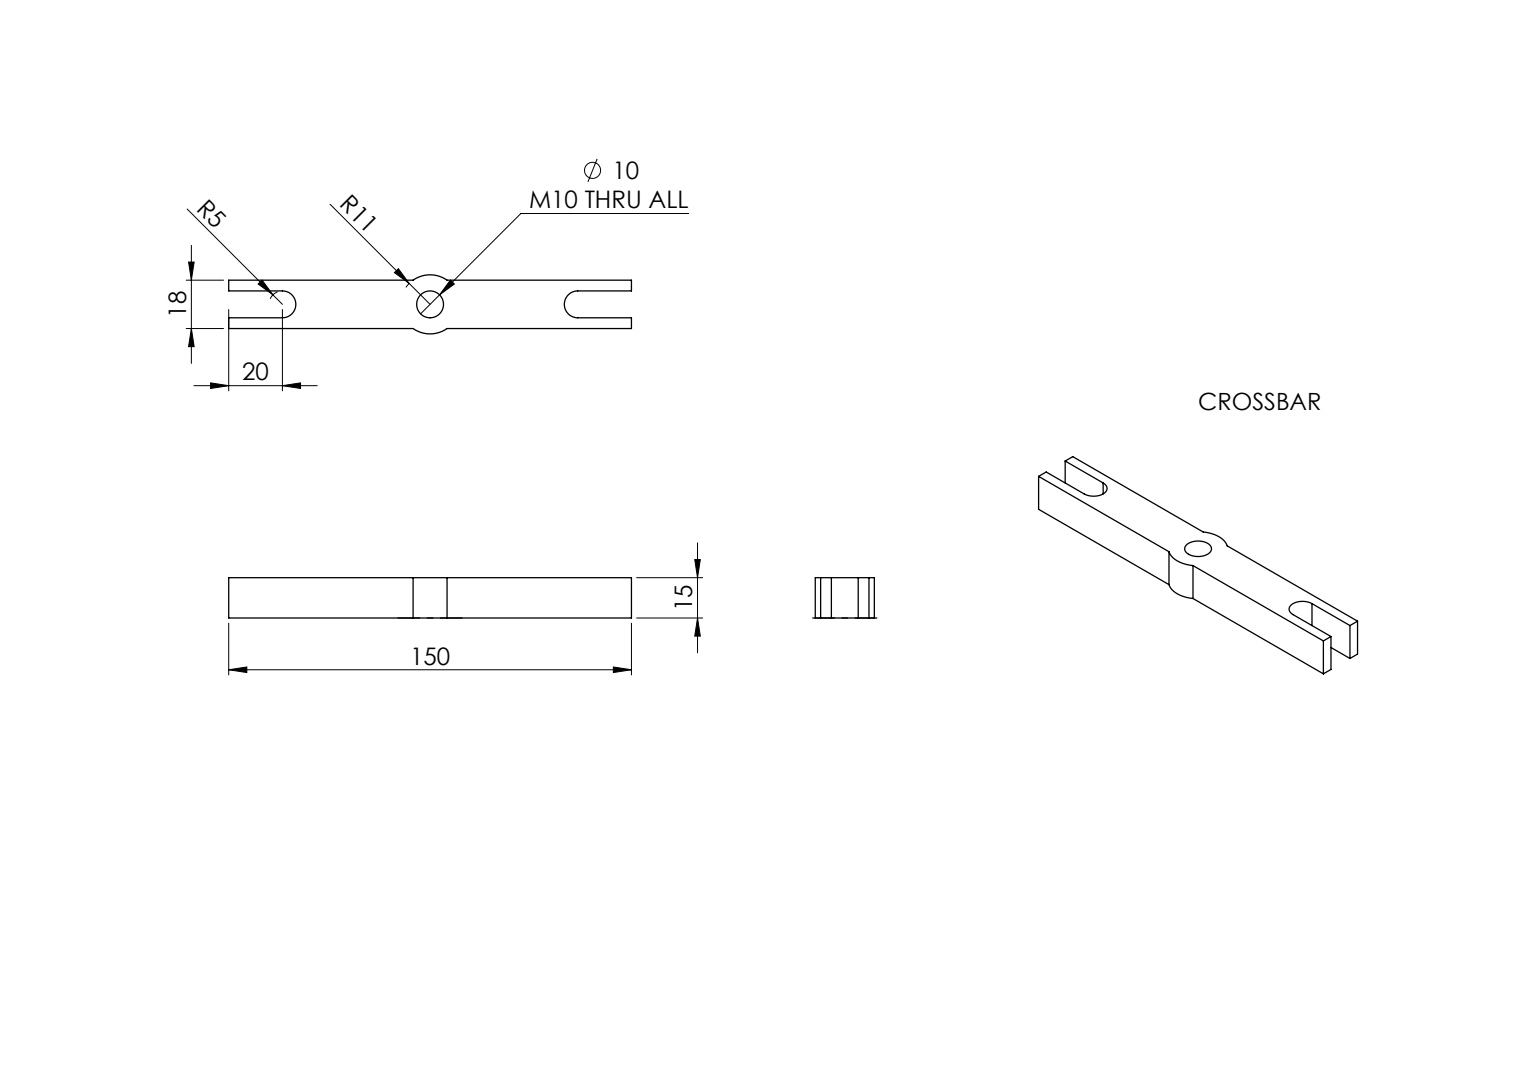
ISO-10303-21;
HEADER;
FILE_DESCRIPTION (('STEP AP214'),
    '1' );
FILE_NAME ('crossbar.step',
    '2026-10-25T05:52:03',
    ( '' ),
    ( '' ),
    'SwSTEP 2.0',
    'SolidWorks 2026',
    '' );
FILE_SCHEMA (( 'AUTOMOTIVE_DESIGN' ));
ENDSEC;

DATA;
#93=MECHANICAL_DESIGN_GEOMETRIC_PRESENTATION_REPRESENTATION('',(#59644),#40104);
#150=CARTESIAN_POINT ( 'NONE',  ( 0.000000000000000000, 15.00000000000000000, 0.000000000000000000 ) ) ;
#164=CARTESIAN_POINT ( 'NONE',  ( 75.00000000000002842, 15.00000000000000000, -5.000000000000000000 ) ) ;
#180=CARTESIAN_POINT ( 'NONE',  ( 75.00000000000000000, 15.00000000000000000, 8.999999999999998224 ) ) ;
#263=ORIENTED_EDGE ( 'NONE', *, *, #11129, .F. ) ;
#343=ORIENTED_EDGE ( 'NONE', *, *, #36170, .F. ) ;
#477=ORIENTED_EDGE ( 'NONE', *, *, #63171, .F. ) ;
#566=PRODUCT_CONTEXT ( 'NONE', #44181, 'mechanical' ) ;
#726=SURFACE_SIDE_STYLE ('',( #44126 ) ) ;
#1131=EDGE_CURVE ( 'NONE', #61397, #19898, #8913, .T. ) ;
#1258=VERTEX_POINT ( 'NONE', #48750 ) ;
#1307=DIRECTION ( 'NONE',  ( 0.000000000000000000, 0.000000000000000000, 1.000000000000000000 ) ) ;
#1344=DIRECTION ( 'NONE',  ( -1.000000000000000000, -0.000000000000000000, -0.000000000000000000 ) ) ;
#1422=LINE ( 'NONE', #21021, #18188 ) ;
#1774=VECTOR ( 'NONE', #54158, 1000.000000000000000 ) ;
#1820=AXIS2_PLACEMENT_3D ( 'NONE', #30255, #49878, #35415 ) ;
#1821=AXIS2_PLACEMENT_3D ( 'NONE', #44111, #19357, #38655 ) ;
#1868=CARTESIAN_POINT ( 'NONE',  ( 75.00000000000002842, 15.00000000000000000, -5.000000000000000000 ) ) ;
#1891=DIRECTION ( 'NONE',  ( -0.000000000000000000, -1.000000000000000000, -0.000000000000000000 ) ) ;
#1911=EDGE_CURVE ( 'NONE', #45549, #35107, #10129, .T. ) ;
#2018=DIRECTION ( 'NONE',  ( 0.000000000000000000, 0.000000000000000000, -1.000000000000000000 ) ) ;
#2144=CARTESIAN_POINT ( 'NONE',  ( 6.324555320336760822, 15.00000000000000000, 8.999999999999998224 ) ) ;
#2154=AXIS2_PLACEMENT_3D ( 'NONE', #31969, #51605, #37127 ) ;
#2168=ORIENTED_EDGE ( 'NONE', *, *, #7515, .F. ) ;
#2189=CARTESIAN_POINT ( 'NONE',  ( -75.00000000000001421, 15.00000000000000000, -9.000000000000001776 ) ) ;
#2419=DIRECTION ( 'NONE',  ( -1.000000000000000000, -0.000000000000000000, -0.000000000000000000 ) ) ;
#2521=EDGE_CURVE ( 'NONE', #37292, #8165, #8808, .T. ) ;
#2523=CARTESIAN_POINT ( 'NONE',  ( 0.000000000000000000, 0.000000000000000000, 0.000000000000000000 ) ) ;
#2751=FACE_OUTER_BOUND ( 'NONE', #28852, .T. ) ;
#3052=DIRECTION ( 'NONE',  ( 1.000000000000000000, -0.000000000000000000, -0.000000000000000000 ) ) ;
#3073=LINE ( 'NONE', #22370, #17419 ) ;
#3217=CARTESIAN_POINT ( 'NONE',  ( -75.00000000000002842, 15.00000000000000000, 5.000000000000000000 ) ) ;
#3275=VECTOR ( 'NONE', #5087, 1000.000000000000000 ) ;
#3526=DIRECTION ( 'NONE',  ( 1.000000000000000000, 0.000000000000000000, 0.000000000000000000 ) ) ;
#3683=LINE ( 'NONE', #52876, #59319 ) ;
#3701=DIRECTION ( 'NONE',  ( 0.000000000000000000, 0.000000000000000000, -1.000000000000000000 ) ) ;
#3724=CARTESIAN_POINT ( 'NONE',  ( 0.000000000000000000, 15.00000000000000000, 0.000000000000000000 ) ) ;
#3861=AXIS2_PLACEMENT_3D ( 'NONE', #23044, #42647, #37831 ) ;
#4005=EDGE_CURVE ( 'NONE', #32177, #5681, #30432, .T. ) ;
#4017=EDGE_CURVE ( 'NONE', #61397, #8313, #22859, .T. ) ;
#4135=VECTOR ( 'NONE', #36854, 1000.000000000000000 ) ;
#4205=ORIENTED_EDGE ( 'NONE', *, *, #4017, .F. ) ;
#4234=PLANE ( 'NONE',  #54494 ) ;
#4424=ORIENTED_EDGE ( 'NONE', *, *, #9501, .T. ) ;
#4477=ORIENTED_EDGE ( 'NONE', *, *, #9853, .F. ) ;
#4648=FACE_OUTER_BOUND ( 'NONE', #37201, .T. ) ;
#4801=ORIENTED_EDGE ( 'NONE', *, *, #10679, .F. ) ;
#5087=DIRECTION ( 'NONE',  ( -1.000000000000000000, -0.000000000000000000, -0.000000000000000000 ) ) ;
#5149=EDGE_CURVE ( 'NONE', #28986, #55261, #41034, .T. ) ;
#5151=CARTESIAN_POINT ( 'NONE',  ( 0.000000000000000000, 15.00000000000000000, 0.000000000000000000 ) ) ;
#5225=AXIS2_PLACEMENT_3D ( 'NONE', #12714, #42297, #61937 ) ;
#5300=CARTESIAN_POINT ( 'NONE',  ( -75.00000000000002842, 15.00000000000000000, -5.000000000000000000 ) ) ;
#5308=VERTEX_POINT ( 'NONE', #62260 ) ;
#5364=EDGE_CURVE ( 'NONE', #32593, #49211, #46190, .T. ) ;
#5608=VECTOR ( 'NONE', #49659, 1000.000000000000000 ) ;
#5626=EDGE_CURVE ( 'NONE', #47522, #36723, #20723, .T. ) ;
#5681=VERTEX_POINT ( 'NONE', #11056 ) ;
#5688=ORIENTED_EDGE ( 'NONE', *, *, #24345, .F. ) ;
#5744=AXIS2_PLACEMENT_3D ( 'NONE', #48462, #49087, #39429 ) ;
#5784=EDGE_LOOP ( 'NONE', ( #54539, #7926, #8477, #60385 ) ) ;
#5805=CARTESIAN_POINT ( 'NONE',  ( -75.00000000000000000, 15.00000000000000000, 8.999999999999998224 ) ) ;
#5822=DIRECTION ( 'NONE',  ( 0.000000000000000000, 0.000000000000000000, 1.000000000000000000 ) ) ;
#5858=EDGE_LOOP ( 'NONE', ( #24339, #2168, #263, #56580 ) ) ;
#5978=VECTOR ( 'NONE', #17876, 1000.000000000000000 ) ;
#6116=AXIS2_PLACEMENT_3D ( 'NONE', #16506, #11988, #35494 ) ;
#6272=EDGE_CURVE ( 'NONE', #47088, #29634, #54076, .T. ) ;
#6365=LINE ( 'NONE', #60400, #57679 ) ;
#6390=LINE ( 'NONE', #55597, #29862 ) ;
#6391=EDGE_LOOP ( 'NONE', ( #33069, #16377, #9474, #4205 ) ) ;
#6429=DIRECTION ( 'NONE',  ( 0.000000000000000000, -1.000000000000000000, 0.000000000000000000 ) ) ;
#6510=DIRECTION ( 'NONE',  ( 0.000000000000000000, -1.000000000000000000, 0.000000000000000000 ) ) ;
#6581=CARTESIAN_POINT ( 'NONE',  ( 75.00000000000002842, 15.00000000000000000, 5.000000000000000000 ) ) ;
#6625=VECTOR ( 'NONE', #29553, 1000.000000000000000 ) ;
#6635=ORIENTED_EDGE ( 'NONE', *, *, #1911, .F. ) ;
#6907=DIRECTION ( 'NONE',  ( -1.000000000000000000, 0.000000000000000000, 0.000000000000000000 ) ) ;
#7158=VERTEX_POINT ( 'NONE', #47572 ) ;
#7165=DIRECTION ( 'NONE',  ( 0.000000000000000000, -1.000000000000000000, 0.000000000000000000 ) ) ;
#7515=EDGE_CURVE ( 'NONE', #8991, #14704, #1422, .T. ) ;
#7900=EDGE_CURVE ( 'NONE', #56115, #33543, #15104, .T. ) ;
#7926=ORIENTED_EDGE ( 'NONE', *, *, #13807, .F. ) ;
#7954=ORIENTED_EDGE ( 'NONE', *, *, #58672, .T. ) ;
#8165=VERTEX_POINT ( 'NONE', #32166 ) ;
#8171=PLANE ( 'NONE',  #2154 ) ;
#8226=DIRECTION ( 'NONE',  ( -1.000000000000000000, 0.000000000000000000, 0.000000000000000000 ) ) ;
#8313=VERTEX_POINT ( 'NONE', #9924 ) ;
#8330=ORIENTED_EDGE ( 'NONE', *, *, #25196, .T. ) ;
#8418=ORIENTED_EDGE ( 'NONE', *, *, #39340, .F. ) ;
#8477=ORIENTED_EDGE ( 'NONE', *, *, #59318, .F. ) ;
#8690=ORIENTED_EDGE ( 'NONE', *, *, #4017, .T. ) ;
#8755=EDGE_LOOP ( 'NONE', ( #42090, #4424, #49121, #32813 ) ) ;
#8808=LINE ( 'NONE', #37769, #20258 ) ;
#8853=FACE_OUTER_BOUND ( 'NONE', #34956, .T. ) ;
#8913=CIRCLE ( 'NONE', #58273, 4.999999999999999112 ) ;
#8991=VERTEX_POINT ( 'NONE', #46151 ) ;
#9169=( GEOMETRIC_REPRESENTATION_CONTEXT ( 3 ) GLOBAL_UNCERTAINTY_ASSIGNED_CONTEXT ( ( #63524 ) ) GLOBAL_UNIT_ASSIGNED_CONTEXT ( ( #59255, #44448, #54100 ) ) REPRESENTATION_CONTEXT ( 'NONE', 'WORKASPACE' ) );
#9174=CIRCLE ( 'NONE', #6116, 5.000000000000000000 ) ;
#9243=LINE ( 'NONE', #18890, #15569 ) ;
#9272=ORIENTED_EDGE ( 'NONE', *, *, #62021, .F. ) ;
#9387=CARTESIAN_POINT ( 'NONE',  ( 6.324555320336760822, 15.00000000000000000, 8.999999999999998224 ) ) ;
#9474=ORIENTED_EDGE ( 'NONE', *, *, #17743, .T. ) ;
#9501=EDGE_CURVE ( 'NONE', #34999, #36723, #10721, .T. ) ;
#9795=CARTESIAN_POINT ( 'NONE',  ( 55.00000000000002132, 15.00000000000000000, 0.000000000000000000 ) ) ;
#9853=EDGE_CURVE ( 'NONE', #24525, #28986, #23225, .T. ) ;
#9872=ORIENTED_EDGE ( 'NONE', *, *, #25196, .F. ) ;
#9924=CARTESIAN_POINT ( 'NONE',  ( 0.000000000000000000, 15.00000000000000000, 5.000000000000000000 ) ) ;
#9961=CARTESIAN_POINT ( 'NONE',  ( 0.000000000000000000, 15.00000000000000000, 0.000000000000000000 ) ) ;
#10016=ADVANCED_FACE ( 'NONE', ( #19653 ), #55032, .F. ) ;
#10039=ORIENTED_EDGE ( 'NONE', *, *, #7515, .T. ) ;
#10087=ORIENTED_EDGE ( 'NONE', *, *, #24861, .T. ) ;
#10109=ORIENTED_EDGE ( 'NONE', *, *, #46867, .F. ) ;
#10129=LINE ( 'NONE', #180, #26454 ) ;
#10143=ORIENTED_EDGE ( 'NONE', *, *, #5626, .T. ) ;
#10259=ORIENTED_EDGE ( 'NONE', *, *, #26003, .T. ) ;
#10412=DIRECTION ( 'NONE',  ( -0.000000000000000000, -1.000000000000000000, -0.000000000000000000 ) ) ;
#10420=CARTESIAN_POINT ( 'NONE',  ( -75.00000000000001421, 15.00000000000000000, -9.000000000000001776 ) ) ;
#10679=EDGE_CURVE ( 'NONE', #57284, #54893, #23658, .T. ) ;
#10721=LINE ( 'NONE', #25513, #27505 ) ;
#10998=ORIENTED_EDGE ( 'NONE', *, *, #18539, .T. ) ;
#11056=CARTESIAN_POINT ( 'NONE',  ( -55.00000000000002132, 15.00000000000000000, -5.000000000000000000 ) ) ;
#11129=EDGE_CURVE ( 'NONE', #1258, #8991, #49113, .T. ) ;
#11150=CIRCLE ( 'NONE', #25528, 5.000000000000000000 ) ;
#11187=DIRECTION ( 'NONE',  ( 0.000000000000000000, -1.000000000000000000, 0.000000000000000000 ) ) ;
#11309=EDGE_LOOP ( 'NONE', ( #34515, #37261, #46350, #54536 ) ) ;
#11440=FACE_OUTER_BOUND ( 'NONE', #51205, .T. ) ;
#11539=DIRECTION ( 'NONE',  ( 0.000000000000000000, 0.000000000000000000, 1.000000000000000000 ) ) ;
#11675=LINE ( 'NONE', #39989, #46329 ) ;
#11732=EDGE_LOOP ( 'NONE', ( #24675, #13816, #20138, #18472 ) ) ;
#11762=ORIENTED_EDGE ( 'NONE', *, *, #2521, .F. ) ;
#11871=LINE ( 'NONE', #56596, #27063 ) ;
#11904=DIRECTION ( 'NONE',  ( -0.000000000000000000, -1.000000000000000000, -0.000000000000000000 ) ) ;
#11910=ADVANCED_FACE ( 'NONE', ( #42379 ), #17315, .T. ) ;
#11988=DIRECTION ( 'NONE',  ( -0.000000000000000000, 1.000000000000000000, -0.000000000000000000 ) ) ;
#12108=FACE_OUTER_BOUND ( 'NONE', #52618, .T. ) ;
#12280=ORIENTED_EDGE ( 'NONE', *, *, #54650, .F. ) ;
#12365=ORIENTED_EDGE ( 'NONE', *, *, #4005, .T. ) ;
#12559=EDGE_CURVE ( 'NONE', #54893, #57064, #27831, .T. ) ;
#12573=DIRECTION ( 'NONE',  ( 0.000000000000000000, 0.000000000000000000, -1.000000000000000000 ) ) ;
#12714=CARTESIAN_POINT ( 'NONE',  ( -55.00000000000002132, 0.000000000000000000, 0.000000000000000000 ) ) ;
#12872=CARTESIAN_POINT ( 'NONE',  ( -55.00000000000002132, 15.00000000000000000, 0.000000000000000000 ) ) ;
#12927=DIRECTION ( 'NONE',  ( 0.000000000000000000, 0.000000000000000000, 1.000000000000000000 ) ) ;
#12975=ORIENTED_EDGE ( 'NONE', *, *, #12559, .F. ) ;
#12976=DIRECTION ( 'NONE',  ( 1.000000000000000000, 0.000000000000000000, 0.000000000000000000 ) ) ;
#13083=ORIENTED_EDGE ( 'NONE', *, *, #55852, .F. ) ;
#13100=( LENGTH_UNIT ( ) NAMED_UNIT ( * ) SI_UNIT ( .MILLI., .METRE. ) );
#13235=CARTESIAN_POINT ( 'NONE',  ( -75.00000000000000000, 0.000000000000000000, 8.999999999999998224 ) ) ;
#13300=ORIENTED_EDGE ( 'NONE', *, *, #7900, .T. ) ;
#13340=PLANE ( 'NONE',  #59479 ) ;
#13356=CARTESIAN_POINT ( 'NONE',  ( -75.00000000000000000, 15.00000000000000000, 8.999999999999998224 ) ) ;
#13468=ADVANCED_FACE ( 'NONE', ( #37030 ), #22874, .T. ) ;
#13484=FACE_BOUND ( 'NONE', #40670, .T. ) ;
#13547=VERTEX_POINT ( 'NONE', #42467 ) ;
#13670=ORIENTED_EDGE ( 'NONE', *, *, #34124, .F. ) ;
#13807=EDGE_CURVE ( 'NONE', #1258, #57064, #57911, .T. ) ;
#13816=ORIENTED_EDGE ( 'NONE', *, *, #5149, .F. ) ;
#13817=DIRECTION ( 'NONE',  ( 0.000000000000000000, 0.000000000000000000, 1.000000000000000000 ) ) ;
#13856=ORIENTED_EDGE ( 'NONE', *, *, #42939, .F. ) ;
#13882=CARTESIAN_POINT ( 'NONE',  ( -75.00000000000000000, 15.00000000000000000, 8.999999999999998224 ) ) ;
#13919=DIRECTION ( 'NONE',  ( 1.000000000000000000, 0.000000000000000000, 0.000000000000000000 ) ) ;
#14074=ORIENTED_EDGE ( 'NONE', *, *, #18539, .F. ) ;
#14144=EDGE_CURVE ( 'NONE', #8313, #16398, #11150, .T. ) ;
#14157=ORIENTED_EDGE ( 'NONE', *, *, #37324, .F. ) ;
#14189=VECTOR ( 'NONE', #3052, 1000.000000000000000 ) ;
#14234=ADVANCED_FACE ( 'NONE', ( #8853 ), #28470, .F. ) ;
#14236=ORIENTED_EDGE ( 'NONE', *, *, #34954, .F. ) ;
#14305=STYLED_ITEM ( 'NONE', ( #19692 ), #24770 ) ;
#14412=DIRECTION ( 'NONE',  ( 0.000000000000000000, -1.000000000000000000, 0.000000000000000000 ) ) ;
#14445=ADVANCED_FACE ( 'NONE', ( #4648 ), #63520, .T. ) ;
#14618=UNCERTAINTY_MEASURE_WITH_UNIT (LENGTH_MEASURE( 1.000000000000000082E-05 ), #20010, 'distance_accuracy_value', 'NONE');
#14661=ORIENTED_EDGE ( 'NONE', *, *, #1911, .T. ) ;
#14704=VERTEX_POINT ( 'NONE', #27767 ) ;
#14783=PRODUCT_DEFINITION_SHAPE ( 'NONE', 'NONE',  #53574 ) ;
#14797=ORIENTED_EDGE ( 'NONE', *, *, #24861, .F. ) ;
#14808=ORIENTED_EDGE ( 'NONE', *, *, #43189, .T. ) ;
#14951=CARTESIAN_POINT ( 'NONE',  ( -55.00000000000002132, 15.00000000000000000, -5.000000000000000000 ) ) ;
#15006=VECTOR ( 'NONE', #3526, 1000.000000000000000 ) ;
#15104=CIRCLE ( 'NONE', #1820, 11.00000000000000000 ) ;
#15481=CARTESIAN_POINT ( 'NONE',  ( 0.000000000000000000, 15.00000000000000000, 0.000000000000000000 ) ) ;
#15569=VECTOR ( 'NONE', #33688, 1000.000000000000000 ) ;
#15748=CARTESIAN_POINT ( 'NONE',  ( -75.00000000000000000, 0.000000000000000000, 8.999999999999998224 ) ) ;
#15753=DIRECTION ( 'NONE',  ( 0.000000000000000000, 1.000000000000000000, 0.000000000000000000 ) ) ;
#15757=ORIENTED_EDGE ( 'NONE', *, *, #54792, .T. ) ;
#15761=EDGE_CURVE ( 'NONE', #55261, #54893, #45335, .T. ) ;
#15836=ORIENTED_EDGE ( 'NONE', *, *, #56237, .F. ) ;
#15970=ORIENTED_EDGE ( 'NONE', *, *, #1131, .T. ) ;
#15986=DIRECTION ( 'NONE',  ( -0.000000000000000000, 1.000000000000000000, -0.000000000000000000 ) ) ;
#16016=CARTESIAN_POINT ( 'NONE',  ( -75.00000000000002842, 15.00000000000000000, -5.000000000000000000 ) ) ;
#16270=PLANE ( 'NONE',  #62054 ) ;
#16377=ORIENTED_EDGE ( 'NONE', *, *, #62021, .T. ) ;
#16398=VERTEX_POINT ( 'NONE', #41056 ) ;
#16506=CARTESIAN_POINT ( 'NONE',  ( 0.000000000000000000, 15.00000000000000000, 0.000000000000000000 ) ) ;
#16597=LINE ( 'NONE', #2144, #4135 ) ;
#16603=DIRECTION ( 'NONE',  ( 7.709882115452476194E-16, 0.000000000000000000, -1.000000000000000000 ) ) ;
#16845=ADVANCED_FACE ( 'NONE', ( #59014 ), #21621, .F. ) ;
#16858=CARTESIAN_POINT ( 'NONE',  ( -6.324555320336756381, 0.000000000000000000, -9.000000000000001776 ) ) ;
#16869=DIRECTION ( 'NONE',  ( 0.000000000000000000, 0.000000000000000000, 1.000000000000000000 ) ) ;
#16955=AXIS2_PLACEMENT_3D ( 'NONE', #37433, #62204, #57065 ) ;
#16959=DIRECTION ( 'NONE',  ( 1.000000000000000000, 0.000000000000000000, -0.000000000000000000 ) ) ;
#17205=EDGE_CURVE ( 'NONE', #57064, #14704, #51349, .T. ) ;
#17257=VERTEX_POINT ( 'NONE', #59804 ) ;
#17315=PLANE ( 'NONE',  #34702 ) ;
#17325=ORIENTED_EDGE ( 'NONE', *, *, #11129, .T. ) ;
#17381=ADVANCED_FACE ( 'NONE', ( #2751 ), #47436, .T. ) ;
#17387=EDGE_CURVE ( 'NONE', #28986, #57284, #3073, .T. ) ;
#17419=VECTOR ( 'NONE', #22690, 1000.000000000000000 ) ;
#17440=ORIENTED_EDGE ( 'NONE', *, *, #59318, .T. ) ;
#17459=VECTOR ( 'NONE', #41732, 1000.000000000000000 ) ;
#17506=CARTESIAN_POINT ( 'NONE',  ( -75.00000000000000000, 0.000000000000000000, 8.999999999999998224 ) ) ;
#17594=VECTOR ( 'NONE', #47304, 1000.000000000000000 ) ;
#17743=EDGE_CURVE ( 'NONE', #16398, #8313, #9174, .T. ) ;
#17751=DIRECTION ( 'NONE',  ( 1.000000000000000000, 0.000000000000000000, 0.000000000000000000 ) ) ;
#17808=CARTESIAN_POINT ( 'NONE',  ( -75.00000000000002842, 15.00000000000000000, 5.000000000000000000 ) ) ;
#17876=DIRECTION ( 'NONE',  ( 7.709882115452476194E-16, 0.000000000000000000, -1.000000000000000000 ) ) ;
#17936=DIRECTION ( 'NONE',  ( 1.000000000000000000, 0.000000000000000000, 0.000000000000000000 ) ) ;
#18188=VECTOR ( 'NONE', #31287, 1000.000000000000000 ) ;
#18368=FACE_OUTER_BOUND ( 'NONE', #11309, .T. ) ;
#18410=VECTOR ( 'NONE', #1344, 1000.000000000000000 ) ;
#18456=AXIS2_PLACEMENT_3D ( 'NONE', #52894, #28127, #3701 ) ;
#18472=ORIENTED_EDGE ( 'NONE', *, *, #10679, .T. ) ;
#18539=EDGE_CURVE ( 'NONE', #17257, #47088, #56236, .T. ) ;
#18621=CARTESIAN_POINT ( 'NONE',  ( -75.00000000000002842, 15.00000000000000000, -5.000000000000000000 ) ) ;
#18677=DIRECTION ( 'NONE',  ( 0.000000000000000000, 0.000000000000000000, -1.000000000000000000 ) ) ;
#18779=DIRECTION ( 'NONE',  ( -1.000000000000000000, 0.000000000000000000, -0.000000000000000000 ) ) ;
#18875=PRODUCT ( 'crossbar', 'crossbar', '', ( #566 ) ) ;
#18890=CARTESIAN_POINT ( 'NONE',  ( -75.00000000000000000, 0.000000000000000000, 8.999999999999998224 ) ) ;
#18963=EDGE_CURVE ( 'NONE', #7158, #24525, #16597, .T. ) ;
#19009=DIRECTION ( 'NONE',  ( 1.000000000000000000, 0.000000000000000000, -0.000000000000000000 ) ) ;
#19045=VECTOR ( 'NONE', #12976, 1000.000000000000000 ) ;
#19129=AXIS2_PLACEMENT_3D ( 'NONE', #2189, #41701, #16959 ) ;
#19188=ORIENTED_EDGE ( 'NONE', *, *, #39340, .T. ) ;
#19357=DIRECTION ( 'NONE',  ( 0.000000000000000000, 0.000000000000000000, -1.000000000000000000 ) ) ;
#19373=( NAMED_UNIT ( * ) PLANE_ANGLE_UNIT ( ) SI_UNIT ( $, .RADIAN. ) );
#19397=ADVANCED_FACE ( 'NONE', ( #29068 ), #59308, .T. ) ;
#19653=FACE_OUTER_BOUND ( 'NONE', #6391, .T. ) ;
#19692=PRESENTATION_STYLE_ASSIGNMENT (( #29653 ) ) ;
#19745=DIRECTION ( 'NONE',  ( -0.000000000000000000, -1.000000000000000000, -0.000000000000000000 ) ) ;
#19765=ORIENTED_EDGE ( 'NONE', *, *, #59330, .T. ) ;
#19793=VERTEX_POINT ( 'NONE', #53451 ) ;
#19898=VERTEX_POINT ( 'NONE', #54409 ) ;
#20010=( LENGTH_UNIT ( ) NAMED_UNIT ( * ) SI_UNIT ( .MILLI., .METRE. ) );
#20138=ORIENTED_EDGE ( 'NONE', *, *, #17387, .T. ) ;
#20258=VECTOR ( 'NONE', #42585, 1000.000000000000000 ) ;
#20336=SHAPE_REPRESENTATION_RELATIONSHIP ( 'NONE' , 'NONE' ,  #21293, #24770 ) ;
#20432=VECTOR ( 'NONE', #6429, 1000.000000000000000 ) ;
#20535=AXIS2_PLACEMENT_3D ( 'NONE', #150, #19745, #58988 ) ;
#20723=LINE ( 'NONE', #10420, #1774 ) ;
#21021=CARTESIAN_POINT ( 'NONE',  ( 55.00000000000002132, 15.00000000000000000, -5.000000000000000000 ) ) ;
#21184=ORIENTED_EDGE ( 'NONE', *, *, #34954, .T. ) ;
#21202=CARTESIAN_POINT ( 'NONE',  ( -75.00000000000000000, 15.00000000000000000, 8.999999999999998224 ) ) ;
#21219=DIRECTION ( 'NONE',  ( 7.709882115452476194E-16, -0.000000000000000000, 1.000000000000000000 ) ) ;
#21287=ORIENTED_EDGE ( 'NONE', *, *, #9501, .F. ) ;
#21293=SHAPE_REPRESENTATION ( 'crossbar', ( #43054 ), #21498 ) ;
#21357=VECTOR ( 'NONE', #6907, 1000.000000000000000 ) ;
#21440=ORIENTED_EDGE ( 'NONE', *, *, #22095, .T. ) ;
#21498=( GEOMETRIC_REPRESENTATION_CONTEXT ( 3 ) GLOBAL_UNCERTAINTY_ASSIGNED_CONTEXT ( ( #14618 ) ) GLOBAL_UNIT_ASSIGNED_CONTEXT ( ( #20010, #19373, #58929 ) ) REPRESENTATION_CONTEXT ( 'NONE', 'WORKASPACE' ) );
#21621=CYLINDRICAL_SURFACE ( 'NONE', #27642, 5.000000000000000000 ) ;
#21637=CARTESIAN_POINT ( 'NONE',  ( -55.00000000000002132, 15.00000000000000000, 5.000000000000000000 ) ) ;
#21838=DIRECTION ( 'NONE',  ( 0.000000000000000000, 1.000000000000000000, 0.000000000000000000 ) ) ;
#21947=ADVANCED_FACE ( 'NONE', ( #11440 ), #55200, .F. ) ;
#21950=FACE_OUTER_BOUND ( 'NONE', #60332, .T. ) ;
#22095=EDGE_CURVE ( 'NONE', #8165, #34549, #56581, .T. ) ;
#22107=PLANE ( 'NONE',  #19129 ) ;
#22137=CARTESIAN_POINT ( 'NONE',  ( -75.00000000000001421, 0.000000000000000000, -9.000000000000001776 ) ) ;
#22211=DIRECTION ( 'NONE',  ( 1.000000000000000000, -0.000000000000000000, -0.000000000000000000 ) ) ;
#22271=DIRECTION ( 'NONE',  ( 0.000000000000000000, -0.000000000000000000, -1.000000000000000000 ) ) ;
#22370=CARTESIAN_POINT ( 'NONE',  ( 75.00000000000000000, 15.00000000000000000, 8.999999999999998224 ) ) ;
#22384=LINE ( 'NONE', #51655, #47156 ) ;
#22390=ORIENTED_EDGE ( 'NONE', *, *, #22398, .T. ) ;
#22398=EDGE_CURVE ( 'NONE', #58460, #19793, #11675, .T. ) ;
#22429=FACE_OUTER_BOUND ( 'NONE', #8755, .T. ) ;
#22558=MECHANICAL_DESIGN_GEOMETRIC_PRESENTATION_REPRESENTATION('',(#14305),#9169);
#22650=LINE ( 'NONE', #17506, #19045 ) ;
#22690=DIRECTION ( 'NONE',  ( -0.000000000000000000, -1.000000000000000000, -0.000000000000000000 ) ) ;
#22831=LINE ( 'NONE', #18621, #3275 ) ;
#22859=LINE ( 'NONE', #27978, #26312 ) ;
#22874=PLANE ( 'NONE',  #53254 ) ;
#22920=FACE_OUTER_BOUND ( 'NONE', #43636, .T. ) ;
#23028=DIRECTION ( 'NONE',  ( -1.000000000000000000, 0.000000000000000000, -0.000000000000000000 ) ) ;
#23044=CARTESIAN_POINT ( 'NONE',  ( 0.000000000000000000, 15.00000000000000000, 0.000000000000000000 ) ) ;
#23071=( NAMED_UNIT ( * ) PLANE_ANGLE_UNIT ( ) SI_UNIT ( $, .RADIAN. ) );
#23225=LINE ( 'NONE', #13882, #34654 ) ;
#23288=VECTOR ( 'NONE', #16603, 1000.000000000000000 ) ;
#23412=CARTESIAN_POINT ( 'NONE',  ( -75.00000000000002842, 15.00000000000000000, -5.000000000000000000 ) ) ;
#23425=VECTOR ( 'NONE', #30375, 1000.000000000000000 ) ;
#23604=AXIS2_PLACEMENT_3D ( 'NONE', #36302, #31786, #45632 ) ;
#23658=LINE ( 'NONE', #62893, #5978 ) ;
#23669=ORIENTED_EDGE ( 'NONE', *, *, #59330, .F. ) ;
#23825=CYLINDRICAL_SURFACE ( 'NONE', #37129, 11.00000000000000000 ) ;
#24247=ORIENTED_EDGE ( 'NONE', *, *, #4005, .F. ) ;
#24339=ORIENTED_EDGE ( 'NONE', *, *, #17205, .T. ) ;
#24345=EDGE_CURVE ( 'NONE', #29634, #34999, #30937, .T. ) ;
#24471=ORIENTED_EDGE ( 'NONE', *, *, #37324, .T. ) ;
#24524=FILL_AREA_STYLE ('',( #58306 ) ) ;
#24525=VERTEX_POINT ( 'NONE', #9387 ) ;
#24675=ORIENTED_EDGE ( 'NONE', *, *, #15761, .F. ) ;
#24770=ADVANCED_BREP_SHAPE_REPRESENTATION ( '', ( #29015, #43054 ), #21498 ) ;
#24861=EDGE_CURVE ( 'NONE', #32177, #8165, #42463, .T. ) ;
#25136=ORIENTED_EDGE ( 'NONE', *, *, #54792, .F. ) ;
#25196=EDGE_CURVE ( 'NONE', #36723, #26676, #9243, .T. ) ;
#25352=CLOSED_SHELL ( 'NONE', ( #10016, #19397, #29448, #21947, #26816, #32085, #40968, #34918, #45695, #28741, #14234, #51439, #17381, #30357, #29838, #44373, #11910, #13468, #16845, #14445, #55014 ) ) ;
#25382=ORIENTED_EDGE ( 'NONE', *, *, #24345, .T. ) ;
#25395=DIRECTION ( 'NONE',  ( 7.709882115452476194E-16, -0.000000000000000000, 1.000000000000000000 ) ) ;
#25404=EDGE_CURVE ( 'NONE', #34999, #13547, #6365, .T. ) ;
#25513=CARTESIAN_POINT ( 'NONE',  ( -75.00000000000001421, 0.000000000000000000, -9.000000000000001776 ) ) ;
#25528=AXIS2_PLACEMENT_3D ( 'NONE', #3724, #31473, #51114 ) ;
#25545=EDGE_LOOP ( 'NONE', ( #15970, #60870 ) ) ;
#25767=CARTESIAN_POINT ( 'NONE',  ( -75.00000000000001421, 15.00000000000000000, -9.000000000000001776 ) ) ;
#26003=EDGE_CURVE ( 'NONE', #35107, #17257, #54196, .T. ) ;
#26125=CARTESIAN_POINT ( 'NONE',  ( 75.00000000000002842, 15.00000000000000000, 5.000000000000000000 ) ) ;
#26184=ORIENTED_EDGE ( 'NONE', *, *, #49243, .T. ) ;
#26236=DIRECTION ( 'NONE',  ( -7.709882115452477180E-16, 0.000000000000000000, 1.000000000000000000 ) ) ;
#26312=VECTOR ( 'NONE', #42768, 1000.000000000000000 ) ;
#26403=VECTOR ( 'NONE', #11904, 1000.000000000000000 ) ;
#26454=VECTOR ( 'NONE', #43579, 1000.000000000000000 ) ;
#26676=VERTEX_POINT ( 'NONE', #27009 ) ;
#26680=PRODUCT_DEFINITION_FORMATION_WITH_SPECIFIED_SOURCE ( 'ANY', '', #18875, .NOT_KNOWN. ) ;
#26771=AXIS2_PLACEMENT_3D ( 'NONE', #30746, #50681, #26236 ) ;
#26806=EDGE_CURVE ( 'NONE', #5681, #42641, #22831, .T. ) ;
#26816=ADVANCED_FACE ( 'NONE', ( #13484, #57865 ), #29511, .F. ) ;
#26860=CARTESIAN_POINT ( 'NONE',  ( -75.00000000000001421, 15.00000000000000000, -9.000000000000001776 ) ) ;
#26967=ORIENTED_EDGE ( 'NONE', *, *, #22095, .F. ) ;
#27004=CARTESIAN_POINT ( 'NONE',  ( 75.00000000000000000, 0.000000000000000000, 8.999999999999998224 ) ) ;
#27009=CARTESIAN_POINT ( 'NONE',  ( -75.00000000000002842, 0.000000000000000000, -5.000000000000000000 ) ) ;
#27063=VECTOR ( 'NONE', #21219, 1000.000000000000000 ) ;
#27084=LINE ( 'NONE', #47953, #42835 ) ;
#27505=VECTOR ( 'NONE', #62939, 1000.000000000000000 ) ;
#27541=VECTOR ( 'NONE', #2419, 1000.000000000000000 ) ;
#27642=AXIS2_PLACEMENT_3D ( 'NONE', #9795, #6510, #2018 ) ;
#27665=DIRECTION ( 'NONE',  ( 0.000000000000000000, 1.000000000000000000, 0.000000000000000000 ) ) ;
#27767=CARTESIAN_POINT ( 'NONE',  ( 55.00000000000002132, -0.000000000000000000, -5.000000000000000000 ) ) ;
#27789=CARTESIAN_POINT ( 'NONE',  ( 75.00000000000002842, 15.00000000000000000, -5.000000000000000000 ) ) ;
#27831=LINE ( 'NONE', #61948, #31682 ) ;
#27978=CARTESIAN_POINT ( 'NONE',  ( 0.000000000000000000, 15.00000000000000000, 4.999999999999999112 ) ) ;
#28127=DIRECTION ( 'NONE',  ( -0.000000000000000000, -1.000000000000000000, -0.000000000000000000 ) ) ;
#28148=VECTOR ( 'NONE', #29409, 1000.000000000000000 ) ;
#28195=CARTESIAN_POINT ( 'NONE',  ( 0.000000000000000000, 0.000000000000000000, 0.000000000000000000 ) ) ;
#28470=PLANE ( 'NONE',  #61499 ) ;
#28704=ORIENTED_EDGE ( 'NONE', *, *, #25404, .T. ) ;
#28741=ADVANCED_FACE ( 'NONE', ( #22920 ), #4234, .F. ) ;
#28773=EDGE_CURVE ( 'NONE', #33543, #29634, #6390, .T. ) ;
#28779=EDGE_LOOP ( 'NONE', ( #11762, #14236, #62039, #10087 ) ) ;
#28838=CYLINDRICAL_SURFACE ( 'NONE', #5744, 5.000000000000000000 ) ;
#28852=EDGE_LOOP ( 'NONE', ( #30021, #31055, #30696, #22390 ) ) ;
#28986=VERTEX_POINT ( 'NONE', #37235 ) ;
#29015=MANIFOLD_SOLID_BREP ( 'AdvancedHole2', #25352 ) ;
#29068=FACE_OUTER_BOUND ( 'NONE', #37644, .T. ) ;
#29262=CARTESIAN_POINT ( 'NONE',  ( 55.00000000000002132, 0.000000000000000000, 5.000000000000000000 ) ) ;
#29409=DIRECTION ( 'NONE',  ( 0.000000000000000000, -1.000000000000000000, 0.000000000000000000 ) ) ;
#29448=ADVANCED_FACE ( 'NONE', ( #40697 ), #16270, .F. ) ;
#29491=CIRCLE ( 'NONE', #3861, 11.00000000000000000 ) ;
#29511=PLANE ( 'NONE',  #55525 ) ;
#29553=DIRECTION ( 'NONE',  ( 1.000000000000000000, 0.000000000000000000, 0.000000000000000000 ) ) ;
#29634=VERTEX_POINT ( 'NONE', #36841 ) ;
#29653=SURFACE_STYLE_USAGE ( .BOTH. , #726 ) ;
#29765=CARTESIAN_POINT ( 'NONE',  ( 75.00000000000000000, 15.00000000000000000, 8.999999999999998224 ) ) ;
#29838=ADVANCED_FACE ( 'NONE', ( #33585 ), #13340, .T. ) ;
#29862=VECTOR ( 'NONE', #1891, 1000.000000000000000 ) ;
#30021=ORIENTED_EDGE ( 'NONE', *, *, #56237, .T. ) ;
#30030=CARTESIAN_POINT ( 'NONE',  ( -75.00000000000000000, 15.00000000000000000, 8.999999999999998224 ) ) ;
#30057=CARTESIAN_POINT ( 'NONE',  ( 75.00000000000002842, 0.000000000000000000, -5.000000000000000000 ) ) ;
#30086=DIRECTION ( 'NONE',  ( -7.709882115452477180E-16, 0.000000000000000000, 1.000000000000000000 ) ) ;
#30255=CARTESIAN_POINT ( 'NONE',  ( 0.000000000000000000, 15.00000000000000000, 0.000000000000000000 ) ) ;
#30291=EDGE_LOOP ( 'NONE', ( #26967, #14797, #12365, #24471 ) ) ;
#30357=ADVANCED_FACE ( 'NONE', ( #18368 ), #23825, .T. ) ;
#30375=DIRECTION ( 'NONE',  ( -1.000000000000000000, -0.000000000000000000, -0.000000000000000000 ) ) ;
#30432=CIRCLE ( 'NONE', #58170, 5.000000000000000000 ) ;
#30576=DIRECTION ( 'NONE',  ( 0.000000000000000000, 0.000000000000000000, 1.000000000000000000 ) ) ;
#30594=ORIENTED_EDGE ( 'NONE', *, *, #55852, .T. ) ;
#30696=ORIENTED_EDGE ( 'NONE', *, *, #43189, .F. ) ;
#30711=DIRECTION ( 'NONE',  ( -0.000000000000000000, -1.000000000000000000, -0.000000000000000000 ) ) ;
#30746=CARTESIAN_POINT ( 'NONE',  ( 75.00000000000000000, 15.00000000000000000, 8.999999999999998224 ) ) ;
#30895=LINE ( 'NONE', #59864, #26403 ) ;
#30937=CIRCLE ( 'NONE', #40212, 11.00000000000000000 ) ;
#31055=ORIENTED_EDGE ( 'NONE', *, *, #18963, .T. ) ;
#31096=DIRECTION ( 'NONE',  ( 0.000000000000000000, 0.000000000000000000, 1.000000000000000000 ) ) ;
#31287=DIRECTION ( 'NONE',  ( 0.000000000000000000, -1.000000000000000000, 0.000000000000000000 ) ) ;
#31466=CARTESIAN_POINT ( 'NONE',  ( 0.000000000000000000, 0.000000000000000000, 0.000000000000000000 ) ) ;
#31473=DIRECTION ( 'NONE',  ( -0.000000000000000000, 1.000000000000000000, -0.000000000000000000 ) ) ;
#31511=EDGE_CURVE ( 'NONE', #8991, #45549, #51929, .T. ) ;
#31636=VECTOR ( 'NONE', #59988, 1000.000000000000000 ) ;
#31642=AXIS2_PLACEMENT_3D ( 'NONE', #48917, #39900, #30576 ) ;
#31676=ORIENTED_EDGE ( 'NONE', *, *, #47226, .F. ) ;
#31682=VECTOR ( 'NONE', #8226, 1000.000000000000000 ) ;
#31786=DIRECTION ( 'NONE',  ( -0.000000000000000000, -1.000000000000000000, -0.000000000000000000 ) ) ;
#31965=ORIENTED_EDGE ( 'NONE', *, *, #42939, .T. ) ;
#31969=CARTESIAN_POINT ( 'NONE',  ( -75.00000000000000000, 15.00000000000000000, 8.999999999999998224 ) ) ;
#32022=ORIENTED_EDGE ( 'NONE', *, *, #31511, .T. ) ;
#32085=ADVANCED_FACE ( 'NONE', ( #61197, #21950 ), #46074, .T. ) ;
#32166=CARTESIAN_POINT ( 'NONE',  ( -55.00000000000002132, 0.000000000000000000, 5.000000000000000000 ) ) ;
#32177=VERTEX_POINT ( 'NONE', #21637 ) ;
#32593=VERTEX_POINT ( 'NONE', #5805 ) ;
#32599=AXIS2_PLACEMENT_3D ( 'NONE', #56755, #56441, #16869 ) ;
#32601=FACE_OUTER_BOUND ( 'NONE', #37600, .T. ) ;
#32813=ORIENTED_EDGE ( 'NONE', *, *, #58672, .F. ) ;
#32979=DIRECTION ( 'NONE',  ( -0.000000000000000000, -1.000000000000000000, -0.000000000000000000 ) ) ;
#33069=ORIENTED_EDGE ( 'NONE', *, *, #61030, .F. ) ;
#33143=ORIENTED_EDGE ( 'NONE', *, *, #36170, .T. ) ;
#33287=DIRECTION ( 'NONE',  ( -0.000000000000000000, 1.000000000000000000, -0.000000000000000000 ) ) ;
#33532=FACE_OUTER_BOUND ( 'NONE', #60854, .T. ) ;
#33543=VERTEX_POINT ( 'NONE', #39297 ) ;
#33585=FACE_OUTER_BOUND ( 'NONE', #28779, .T. ) ;
#33603=ORIENTED_EDGE ( 'NONE', *, *, #26806, .T. ) ;
#33670=FACE_OUTER_BOUND ( 'NONE', #30291, .T. ) ;
#33688=DIRECTION ( 'NONE',  ( 7.709882115452476194E-16, -0.000000000000000000, 1.000000000000000000 ) ) ;
#33911=VECTOR ( 'NONE', #30711, 1000.000000000000000 ) ;
#34078=DIRECTION ( 'NONE',  ( 0.000000000000000000, -1.000000000000000000, 0.000000000000000000 ) ) ;
#34124=EDGE_CURVE ( 'NONE', #37292, #49211, #34724, .T. ) ;
#34233=CARTESIAN_POINT ( 'NONE',  ( -55.00000000000002132, 0.000000000000000000, -5.000000000000000000 ) ) ;
#34345=CARTESIAN_POINT ( 'NONE',  ( 0.000000000000000000, 15.00000000000000000, 0.000000000000000000 ) ) ;
#34515=ORIENTED_EDGE ( 'NONE', *, *, #28773, .F. ) ;
#34549=VERTEX_POINT ( 'NONE', #34233 ) ;
#34650=CIRCLE ( 'NONE', #32599, 11.00000000000000000 ) ;
#34654=VECTOR ( 'NONE', #57340, 1000.000000000000000 ) ;
#34702=AXIS2_PLACEMENT_3D ( 'NONE', #23412, #62656, #17936 ) ;
#34724=LINE ( 'NONE', #15748, #45142 ) ;
#34884=DIRECTION ( 'NONE',  ( 0.000000000000000000, 0.000000000000000000, 1.000000000000000000 ) ) ;
#34900=CARTESIAN_POINT ( 'NONE',  ( -75.00000000000002842, 0.000000000000000000, 5.000000000000000000 ) ) ;
#34918=ADVANCED_FACE ( 'NONE', ( #32601 ), #8171, .F. ) ;
#34954=EDGE_CURVE ( 'NONE', #5308, #37292, #51291, .T. ) ;
#34956=EDGE_LOOP ( 'NONE', ( #45657, #31965, #55754, #4477 ) ) ;
#34999=VERTEX_POINT ( 'NONE', #16858 ) ;
#35107=VERTEX_POINT ( 'NONE', #57690 ) ;
#35367=CARTESIAN_POINT ( 'NONE',  ( 75.00000000000002842, 15.00000000000000000, 5.000000000000000000 ) ) ;
#35415=DIRECTION ( 'NONE',  ( 0.000000000000000000, 0.000000000000000000, 1.000000000000000000 ) ) ;
#35494=DIRECTION ( 'NONE',  ( 0.000000000000000000, 0.000000000000000000, 1.000000000000000000 ) ) ;
#35824=AXIS2_PLACEMENT_3D ( 'NONE', #164, #34884, #54506 ) ;
#35889=DIRECTION ( 'NONE',  ( -1.000000000000000000, 0.000000000000000000, -7.709882115452477180E-16 ) ) ;
#36159=ORIENTED_EDGE ( 'NONE', *, *, #59338, .F. ) ;
#36170=EDGE_CURVE ( 'NONE', #5308, #32593, #11871, .T. ) ;
#36302=CARTESIAN_POINT ( 'NONE',  ( 55.00000000000002132, 0.000000000000000000, 0.000000000000000000 ) ) ;
#36422=CARTESIAN_POINT ( 'NONE',  ( 0.000000000000000000, 0.000000000000000000, 0.000000000000000000 ) ) ;
#36508=CIRCLE ( 'NONE', #45742, 11.00000000000000000 ) ;
#36584=CARTESIAN_POINT ( 'NONE',  ( -75.00000000000001421, 15.00000000000000000, -9.000000000000001776 ) ) ;
#36723=VERTEX_POINT ( 'NONE', #59107 ) ;
#36779=CARTESIAN_POINT ( 'NONE',  ( 0.000000000000000000, 0.000000000000000000, 0.000000000000000000 ) ) ;
#36841=CARTESIAN_POINT ( 'NONE',  ( 0.000000000000000000, 0.000000000000000000, -11.00000000000000000 ) ) ;
#36854=DIRECTION ( 'NONE',  ( 0.000000000000000000, 1.000000000000000000, 0.000000000000000000 ) ) ;
#36920=COLOUR_RGB ( '',0.8941176470588234615, 0.8941176470588234615, 0.8941176470588234615 ) ;
#37030=FACE_OUTER_BOUND ( 'NONE', #5784, .T. ) ;
#37106=DIRECTION ( 'NONE',  ( 0.000000000000000000, 0.000000000000000000, 1.000000000000000000 ) ) ;
#37127=DIRECTION ( 'NONE',  ( -7.709882115452477180E-16, 0.000000000000000000, -1.000000000000000000 ) ) ;
#37129=AXIS2_PLACEMENT_3D ( 'NONE', #5151, #43117, #18677 ) ;
#37201=EDGE_LOOP ( 'NONE', ( #15757, #47096, #53948, #10039 ) ) ;
#37235=CARTESIAN_POINT ( 'NONE',  ( 75.00000000000000000, 15.00000000000000000, 8.999999999999998224 ) ) ;
#37261=ORIENTED_EDGE ( 'NONE', *, *, #7900, .F. ) ;
#37292=VERTEX_POINT ( 'NONE', #34900 ) ;
#37324=EDGE_CURVE ( 'NONE', #5681, #34549, #58704, .T. ) ;
#37433=CARTESIAN_POINT ( 'NONE',  ( -75.00000000000000000, 15.00000000000000000, 8.999999999999998224 ) ) ;
#37434=DIRECTION ( 'NONE',  ( 0.000000000000000000, -1.000000000000000000, 0.000000000000000000 ) ) ;
#37600=EDGE_LOOP ( 'NONE', ( #31676, #8418, #10143, #8330 ) ) ;
#37644=EDGE_LOOP ( 'NONE', ( #13083, #54570, #25382, #28704 ) ) ;
#37769=CARTESIAN_POINT ( 'NONE',  ( -75.00000000000002842, 0.000000000000000000, 5.000000000000000000 ) ) ;
#37789=DIRECTION ( 'NONE',  ( 0.000000000000000000, 0.000000000000000000, -1.000000000000000000 ) ) ;
#37831=DIRECTION ( 'NONE',  ( 0.000000000000000000, 0.000000000000000000, 1.000000000000000000 ) ) ;
#37833=AXIS2_PLACEMENT_3D ( 'NONE', #2523, #50458, #45300 ) ;
#37891=EDGE_LOOP ( 'NONE', ( #21184, #51187, #45835, #343 ) ) ;
#38367=DIRECTION ( 'NONE',  ( 0.000000000000000000, 0.000000000000000000, 1.000000000000000000 ) ) ;
#38379=ORIENTED_EDGE ( 'NONE', *, *, #17743, .F. ) ;
#38655=DIRECTION ( 'NONE',  ( -1.000000000000000000, 0.000000000000000000, -0.000000000000000000 ) ) ;
#38870=VECTOR ( 'NONE', #34078, 1000.000000000000000 ) ;
#39045=LINE ( 'NONE', #30030, #5608 ) ;
#39208=CARTESIAN_POINT ( 'NONE',  ( -75.00000000000000000, 15.00000000000000000, 8.999999999999998224 ) ) ;
#39297=CARTESIAN_POINT ( 'NONE',  ( 0.000000000000000000, 15.00000000000000000, -11.00000000000000000 ) ) ;
#39340=EDGE_CURVE ( 'NONE', #47522, #42641, #39045, .T. ) ;
#39387=CARTESIAN_POINT ( 'NONE',  ( 6.324555320336756381, 15.00000000000000000, -9.000000000000001776 ) ) ;
#39429=DIRECTION ( 'NONE',  ( 0.000000000000000000, 0.000000000000000000, -1.000000000000000000 ) ) ;
#39449=ORIENTED_EDGE ( 'NONE', *, *, #2521, .T. ) ;
#39474=ORIENTED_EDGE ( 'NONE', *, *, #14144, .T. ) ;
#39588=ORIENTED_EDGE ( 'NONE', *, *, #59338, .T. ) ;
#39900=DIRECTION ( 'NONE',  ( -0.000000000000000000, -1.000000000000000000, -0.000000000000000000 ) ) ;
#39989=CARTESIAN_POINT ( 'NONE',  ( -6.324555320336760822, 15.00000000000000000, 8.999999999999998224 ) ) ;
#40098=SHAPE_DEFINITION_REPRESENTATION ( #14783, #21293 ) ;
#40104=( GEOMETRIC_REPRESENTATION_CONTEXT ( 3 ) GLOBAL_UNCERTAINTY_ASSIGNED_CONTEXT ( ( #43308 ) ) GLOBAL_UNIT_ASSIGNED_CONTEXT ( ( #13100, #23071, #61061 ) ) REPRESENTATION_CONTEXT ( 'NONE', 'WORKASPACE' ) );
#40212=AXIS2_PLACEMENT_3D ( 'NONE', #36779, #56412, #37106 ) ;
#40308=EDGE_CURVE ( 'NONE', #32593, #58460, #49503, .T. ) ;
#40346=CARTESIAN_POINT ( 'NONE',  ( 75.00000000000000000, 0.000000000000000000, 8.999999999999998224 ) ) ;
#40670=EDGE_LOOP ( 'NONE', ( #51492, #38379 ) ) ;
#40697=FACE_OUTER_BOUND ( 'NONE', #11732, .T. ) ;
#40715=ORIENTED_EDGE ( 'NONE', *, *, #9853, .T. ) ;
#40968=ADVANCED_FACE ( 'NONE', ( #50960 ), #61891, .F. ) ;
#41034=LINE ( 'NONE', #60681, #23288 ) ;
#41056=CARTESIAN_POINT ( 'NONE',  ( 6.123233995736766282E-16, 15.00000000000000000, -5.000000000000000000 ) ) ;
#41198=CARTESIAN_POINT ( 'NONE',  ( 75.00000000000002842, 15.00000000000000000, 5.000000000000000000 ) ) ;
#41509=CARTESIAN_POINT ( 'NONE',  ( -55.00000000000002132, 15.00000000000000000, 5.000000000000000000 ) ) ;
#41513=DIRECTION ( 'NONE',  ( 1.000000000000000000, 0.000000000000000000, 0.000000000000000000 ) ) ;
#41606=CARTESIAN_POINT ( 'NONE',  ( -75.00000000000002842, 0.000000000000000000, -5.000000000000000000 ) ) ;
#41701=DIRECTION ( 'NONE',  ( 0.000000000000000000, 0.000000000000000000, 1.000000000000000000 ) ) ;
#41732=DIRECTION ( 'NONE',  ( -1.000000000000000000, -0.000000000000000000, -0.000000000000000000 ) ) ;
#41852=ORIENTED_EDGE ( 'NONE', *, *, #1131, .F. ) ;
#42090=ORIENTED_EDGE ( 'NONE', *, *, #25404, .F. ) ;
#42297=DIRECTION ( 'NONE',  ( 0.000000000000000000, 1.000000000000000000, 0.000000000000000000 ) ) ;
#42379=FACE_OUTER_BOUND ( 'NONE', #54402, .T. ) ;
#42463=LINE ( 'NONE', #41509, #17594 ) ;
#42467=CARTESIAN_POINT ( 'NONE',  ( -6.324555320336756381, 15.00000000000000000, -9.000000000000001776 ) ) ;
#42585=DIRECTION ( 'NONE',  ( 1.000000000000000000, 0.000000000000000000, 0.000000000000000000 ) ) ;
#42586=LINE ( 'NONE', #26860, #27541 ) ;
#42641=VERTEX_POINT ( 'NONE', #5300 ) ;
#42647=DIRECTION ( 'NONE',  ( 0.000000000000000000, 1.000000000000000000, 0.000000000000000000 ) ) ;
#42768=DIRECTION ( 'NONE',  ( -0.000000000000000000, 1.000000000000000000, -0.000000000000000000 ) ) ;
#42835=VECTOR ( 'NONE', #17751, 1000.000000000000000 ) ;
#42939=EDGE_CURVE ( 'NONE', #7158, #57284, #22650, .T. ) ;
#42985=AXIS2_PLACEMENT_3D ( 'NONE', #36422, #7165, #22271 ) ;
#42991=DIRECTION ( 'NONE',  ( 0.000000000000000000, 0.000000000000000000, 1.000000000000000000 ) ) ;
#43054=AXIS2_PLACEMENT_3D ( 'NONE', #62200, #38367, #13919 ) ;
#43058=DIRECTION ( 'NONE',  ( 0.000000000000000000, -0.000000000000000000, -1.000000000000000000 ) ) ;
#43117=DIRECTION ( 'NONE',  ( -0.000000000000000000, -1.000000000000000000, -0.000000000000000000 ) ) ;
#43189=EDGE_CURVE ( 'NONE', #58460, #24525, #36508, .T. ) ;
#43308=UNCERTAINTY_MEASURE_WITH_UNIT (LENGTH_MEASURE( 1.000000000000000082E-05 ), #13100, 'distance_accuracy_value', 'NONE');
#43316=CARTESIAN_POINT ( 'NONE',  ( 0.000000000000000000, 0.000000000000000000, 4.999999999999999112 ) ) ;
#43466=ORIENTED_EDGE ( 'NONE', *, *, #40308, .T. ) ;
#43579=DIRECTION ( 'NONE',  ( 7.709882115452476194E-16, 0.000000000000000000, -1.000000000000000000 ) ) ;
#43636=EDGE_LOOP ( 'NONE', ( #12280, #477, #10259, #10998 ) ) ;
#44111=CARTESIAN_POINT ( 'NONE',  ( -75.00000000000000000, 15.00000000000000000, 8.999999999999998224 ) ) ;
#44126=SURFACE_STYLE_FILL_AREA ( #24524 ) ;
#44181=APPLICATION_CONTEXT ( 'automotive_design' ) ;
#44373=ADVANCED_FACE ( 'NONE', ( #33670 ), #28838, .F. ) ;
#44448=( NAMED_UNIT ( * ) PLANE_ANGLE_UNIT ( ) SI_UNIT ( $, .RADIAN. ) );
#45142=VECTOR ( 'NONE', #25395, 1000.000000000000000 ) ;
#45300=DIRECTION ( 'NONE',  ( 0.000000000000000000, 0.000000000000000000, 1.000000000000000000 ) ) ;
#45335=LINE ( 'NONE', #35367, #20432 ) ;
#45511=CARTESIAN_POINT ( 'NONE',  ( -6.324555320336760822, 15.00000000000000000, 8.999999999999998224 ) ) ;
#45549=VERTEX_POINT ( 'NONE', #1868 ) ;
#45632=DIRECTION ( 'NONE',  ( 0.000000000000000000, 0.000000000000000000, 1.000000000000000000 ) ) ;
#45657=ORIENTED_EDGE ( 'NONE', *, *, #18963, .F. ) ;
#45695=ADVANCED_FACE ( 'NONE', ( #22429 ), #22107, .F. ) ;
#45742=AXIS2_PLACEMENT_3D ( 'NONE', #9961, #15753, #1307 ) ;
#45835=ORIENTED_EDGE ( 'NONE', *, *, #5364, .F. ) ;
#45890=CARTESIAN_POINT ( 'NONE',  ( 0.000000000000000000, 15.00000000000000000, 0.000000000000000000 ) ) ;
#46059=ORIENTED_EDGE ( 'NONE', *, *, #50433, .T. ) ;
#46074=PLANE ( 'NONE',  #42985 ) ;
#46151=CARTESIAN_POINT ( 'NONE',  ( 55.00000000000002132, 15.00000000000000000, -5.000000000000000000 ) ) ;
#46190=LINE ( 'NONE', #13356, #59229 ) ;
#46329=VECTOR ( 'NONE', #10412, 1000.000000000000000 ) ;
#46350=ORIENTED_EDGE ( 'NONE', *, *, #54650, .T. ) ;
#46556=DIRECTION ( 'NONE',  ( 0.000000000000000000, -1.000000000000000000, 0.000000000000000000 ) ) ;
#46601=DIRECTION ( 'NONE',  ( 0.000000000000000000, 0.000000000000000000, -1.000000000000000000 ) ) ;
#46867=EDGE_CURVE ( 'NONE', #5308, #32177, #61124, .T. ) ;
#47088=VERTEX_POINT ( 'NONE', #58495 ) ;
#47096=ORIENTED_EDGE ( 'NONE', *, *, #50433, .F. ) ;
#47156=VECTOR ( 'NONE', #33287, 1000.000000000000000 ) ;
#47226=EDGE_CURVE ( 'NONE', #42641, #26676, #55588, .T. ) ;
#47304=DIRECTION ( 'NONE',  ( 0.000000000000000000, -1.000000000000000000, 0.000000000000000000 ) ) ;
#47436=CYLINDRICAL_SURFACE ( 'NONE', #18456, 11.00000000000000000 ) ;
#47522=VERTEX_POINT ( 'NONE', #36584 ) ;
#47572=CARTESIAN_POINT ( 'NONE',  ( 6.324555320336760822, 0.000000000000000000, 8.999999999999998224 ) ) ;
#47810=DIRECTION ( 'NONE',  ( -0.000000000000000000, 1.000000000000000000, -0.000000000000000000 ) ) ;
#47953=CARTESIAN_POINT ( 'NONE',  ( -75.00000000000000000, 0.000000000000000000, 8.999999999999998224 ) ) ;
#48462=CARTESIAN_POINT ( 'NONE',  ( -55.00000000000002132, 15.00000000000000000, 0.000000000000000000 ) ) ;
#48555=CARTESIAN_POINT ( 'NONE',  ( 55.00000000000002132, 15.00000000000000000, 5.000000000000000000 ) ) ;
#48689=APPLICATION_CONTEXT ( 'automotive_design' ) ;
#48750=CARTESIAN_POINT ( 'NONE',  ( 55.00000000000002132, 15.00000000000000000, 5.000000000000000000 ) ) ;
#48917=CARTESIAN_POINT ( 'NONE',  ( 55.00000000000002132, 15.00000000000000000, 0.000000000000000000 ) ) ;
#49087=DIRECTION ( 'NONE',  ( 0.000000000000000000, -1.000000000000000000, 0.000000000000000000 ) ) ;
#49108=CIRCLE ( 'NONE', #37833, 4.999999999999999112 ) ;
#49113=CIRCLE ( 'NONE', #31642, 5.000000000000000000 ) ;
#49121=ORIENTED_EDGE ( 'NONE', *, *, #5626, .F. ) ;
#49211=VERTEX_POINT ( 'NONE', #13235 ) ;
#49243=EDGE_CURVE ( 'NONE', #49211, #19793, #27084, .T. ) ;
#49503=LINE ( 'NONE', #39208, #6625 ) ;
#49659=DIRECTION ( 'NONE',  ( 7.709882115452476194E-16, -0.000000000000000000, 1.000000000000000000 ) ) ;
#49878=DIRECTION ( 'NONE',  ( 0.000000000000000000, 1.000000000000000000, 0.000000000000000000 ) ) ;
#49998=LINE ( 'NONE', #40346, #31636 ) ;
#50041=VECTOR ( 'NONE', #22211, 1000.000000000000000 ) ;
#50089=AXIS2_PLACEMENT_3D ( 'NONE', #15481, #59872, #5822 ) ;
#50092=DIRECTION ( 'NONE',  ( 0.000000000000000000, 1.000000000000000000, 0.000000000000000000 ) ) ;
#50433=EDGE_CURVE ( 'NONE', #45549, #55857, #3683, .T. ) ;
#50458=DIRECTION ( 'NONE',  ( -0.000000000000000000, 1.000000000000000000, -0.000000000000000000 ) ) ;
#50491=ORIENTED_EDGE ( 'NONE', *, *, #26003, .F. ) ;
#50681=DIRECTION ( 'NONE',  ( -1.000000000000000000, 0.000000000000000000, -7.709882115452477180E-16 ) ) ;
#50960=FACE_OUTER_BOUND ( 'NONE', #37891, .T. ) ;
#51114=DIRECTION ( 'NONE',  ( 0.000000000000000000, 0.000000000000000000, 1.000000000000000000 ) ) ;
#51187=ORIENTED_EDGE ( 'NONE', *, *, #34124, .T. ) ;
#51205=EDGE_LOOP ( 'NONE', ( #46059, #39588, #50491, #6635 ) ) ;
#51291=LINE ( 'NONE', #17808, #62743 ) ;
#51294=LINE ( 'NONE', #41606, #23425 ) ;
#51349=CIRCLE ( 'NONE', #23604, 5.000000000000000000 ) ;
#51439=ADVANCED_FACE ( 'NONE', ( #33532 ), #53147, .F. ) ;
#51492=ORIENTED_EDGE ( 'NONE', *, *, #14144, .F. ) ;
#51605=DIRECTION ( 'NONE',  ( 1.000000000000000000, 0.000000000000000000, -7.709882115452477180E-16 ) ) ;
#51655=CARTESIAN_POINT ( 'NONE',  ( 6.123233995736765296E-16, 15.00000000000000000, -4.999999999999999112 ) ) ;
#51877=ORIENTED_EDGE ( 'NONE', *, *, #49243, .F. ) ;
#51929=LINE ( 'NONE', #27789, #14189 ) ;
#52108=CARTESIAN_POINT ( 'NONE',  ( 75.00000000000002842, 0.000000000000000000, 5.000000000000000000 ) ) ;
#52618=EDGE_LOOP ( 'NONE', ( #9272, #41852, #8690, #39474 ) ) ;
#52876=CARTESIAN_POINT ( 'NONE',  ( 75.00000000000002842, 15.00000000000000000, -5.000000000000000000 ) ) ;
#52894=CARTESIAN_POINT ( 'NONE',  ( 0.000000000000000000, 15.00000000000000000, 0.000000000000000000 ) ) ;
#52897=ORIENTED_EDGE ( 'NONE', *, *, #5149, .T. ) ;
#53075=AXIS2_PLACEMENT_3D ( 'NONE', #31466, #21838, #11539 ) ;
#53147=PLANE ( 'NONE',  #1821 ) ;
#53254=AXIS2_PLACEMENT_3D ( 'NONE', #41198, #12573, #41513 ) ;
#53451=CARTESIAN_POINT ( 'NONE',  ( -6.324555320336760822, 0.000000000000000000, 8.999999999999998224 ) ) ;
#53558=ORIENTED_EDGE ( 'NONE', *, *, #26806, .F. ) ;
#53574=PRODUCT_DEFINITION ( 'UNKNOWN', '', #26680, #63075 ) ;
#53879=CARTESIAN_POINT ( 'NONE',  ( 75.00000000000001421, 15.00000000000000000, -9.000000000000001776 ) ) ;
#53948=ORIENTED_EDGE ( 'NONE', *, *, #31511, .F. ) ;
#54076=CIRCLE ( 'NONE', #53075, 11.00000000000000000 ) ;
#54100=( NAMED_UNIT ( * ) SI_UNIT ( $, .STERADIAN. ) SOLID_ANGLE_UNIT ( ) );
#54158=DIRECTION ( 'NONE',  ( -0.000000000000000000, -1.000000000000000000, -0.000000000000000000 ) ) ;
#54196=LINE ( 'NONE', #53879, #33911 ) ;
#54402=EDGE_LOOP ( 'NONE', ( #23669, #14157, #33603, #58373 ) ) ;
#54409=CARTESIAN_POINT ( 'NONE',  ( 6.123233995736765296E-16, 0.000000000000000000, -4.999999999999999112 ) ) ;
#54440=ORIENTED_EDGE ( 'NONE', *, *, #5364, .T. ) ;
#54494=AXIS2_PLACEMENT_3D ( 'NONE', #63097, #12927, #19009 ) ;
#54506=DIRECTION ( 'NONE',  ( -1.000000000000000000, 0.000000000000000000, 0.000000000000000000 ) ) ;
#54536=ORIENTED_EDGE ( 'NONE', *, *, #6272, .T. ) ;
#54539=ORIENTED_EDGE ( 'NONE', *, *, #12559, .T. ) ;
#54570=ORIENTED_EDGE ( 'NONE', *, *, #28773, .T. ) ;
#54650=EDGE_CURVE ( 'NONE', #56115, #47088, #30895, .T. ) ;
#54719=LINE ( 'NONE', #25767, #18410 ) ;
#54792=EDGE_CURVE ( 'NONE', #14704, #55857, #57577, .T. ) ;
#54893=VERTEX_POINT ( 'NONE', #52108 ) ;
#55014=ADVANCED_FACE ( 'NONE', ( #12108 ), #55873, .F. ) ;
#55032=CYLINDRICAL_SURFACE ( 'NONE', #50089, 4.999999999999999112 ) ;
#55156=VECTOR ( 'NONE', #11187, 1000.000000000000000 ) ;
#55158=LINE ( 'NONE', #6581, #21357 ) ;
#55200=PLANE ( 'NONE',  #26771 ) ;
#55261=VERTEX_POINT ( 'NONE', #26125 ) ;
#55525=AXIS2_PLACEMENT_3D ( 'NONE', #34345, #14412, #43058 ) ;
#55588=LINE ( 'NONE', #16016, #55156 ) ;
#55597=CARTESIAN_POINT ( 'NONE',  ( 0.000000000000000000, 15.00000000000000000, -11.00000000000000000 ) ) ;
#55754=ORIENTED_EDGE ( 'NONE', *, *, #17387, .F. ) ;
#55852=EDGE_CURVE ( 'NONE', #33543, #13547, #29491, .T. ) ;
#55857=VERTEX_POINT ( 'NONE', #30057 ) ;
#55873=CYLINDRICAL_SURFACE ( 'NONE', #59268, 4.999999999999999112 ) ;
#56115=VERTEX_POINT ( 'NONE', #39387 ) ;
#56236=LINE ( 'NONE', #22137, #17459 ) ;
#56237=EDGE_CURVE ( 'NONE', #19793, #7158, #34650, .T. ) ;
#56412=DIRECTION ( 'NONE',  ( 0.000000000000000000, 1.000000000000000000, 0.000000000000000000 ) ) ;
#56441=DIRECTION ( 'NONE',  ( 0.000000000000000000, 1.000000000000000000, 0.000000000000000000 ) ) ;
#56580=ORIENTED_EDGE ( 'NONE', *, *, #13807, .T. ) ;
#56581=CIRCLE ( 'NONE', #5225, 5.000000000000000000 ) ;
#56596=CARTESIAN_POINT ( 'NONE',  ( -75.00000000000000000, 15.00000000000000000, 8.999999999999998224 ) ) ;
#56755=CARTESIAN_POINT ( 'NONE',  ( 0.000000000000000000, 0.000000000000000000, 0.000000000000000000 ) ) ;
#57064=VERTEX_POINT ( 'NONE', #29262 ) ;
#57065=DIRECTION ( 'NONE',  ( -7.709882115452477180E-16, 0.000000000000000000, -1.000000000000000000 ) ) ;
#57133=ORIENTED_EDGE ( 'NONE', *, *, #40308, .F. ) ;
#57284=VERTEX_POINT ( 'NONE', #27004 ) ;
#57340=DIRECTION ( 'NONE',  ( 1.000000000000000000, 0.000000000000000000, 0.000000000000000000 ) ) ;
#57371=ORIENTED_EDGE ( 'NONE', *, *, #63171, .T. ) ;
#57577=LINE ( 'NONE', #61454, #50041 ) ;
#57679=VECTOR ( 'NONE', #50092, 1000.000000000000000 ) ;
#57690=CARTESIAN_POINT ( 'NONE',  ( 75.00000000000001421, 15.00000000000000000, -9.000000000000001776 ) ) ;
#57732=ORIENTED_EDGE ( 'NONE', *, *, #22398, .F. ) ;
#57865=FACE_OUTER_BOUND ( 'NONE', #61961, .T. ) ;
#57911=LINE ( 'NONE', #48555, #38870 ) ;
#58170=AXIS2_PLACEMENT_3D ( 'NONE', #12872, #27665, #13817 ) ;
#58204=ORIENTED_EDGE ( 'NONE', *, *, #17205, .F. ) ;
#58273=AXIS2_PLACEMENT_3D ( 'NONE', #28195, #47810, #42991 ) ;
#58306=FILL_AREA_STYLE_COLOUR ( '', #36920 ) ;
#58373=ORIENTED_EDGE ( 'NONE', *, *, #47226, .T. ) ;
#58460=VERTEX_POINT ( 'NONE', #45511 ) ;
#58495=CARTESIAN_POINT ( 'NONE',  ( 6.324555320336756381, 0.000000000000000000, -9.000000000000001776 ) ) ;
#58672=EDGE_CURVE ( 'NONE', #13547, #47522, #42586, .T. ) ;
#58704=LINE ( 'NONE', #14951, #28148 ) ;
#58929=( NAMED_UNIT ( * ) SI_UNIT ( $, .STERADIAN. ) SOLID_ANGLE_UNIT ( ) );
#58988=DIRECTION ( 'NONE',  ( 0.000000000000000000, 0.000000000000000000, -1.000000000000000000 ) ) ;
#59014=FACE_OUTER_BOUND ( 'NONE', #5858, .T. ) ;
#59107=CARTESIAN_POINT ( 'NONE',  ( -75.00000000000001421, 0.000000000000000000, -9.000000000000001776 ) ) ;
#59229=VECTOR ( 'NONE', #32979, 1000.000000000000000 ) ;
#59255=( LENGTH_UNIT ( ) NAMED_UNIT ( * ) SI_UNIT ( .MILLI., .METRE. ) );
#59268=AXIS2_PLACEMENT_3D ( 'NONE', #45890, #15986, #31096 ) ;
#59308=CYLINDRICAL_SURFACE ( 'NONE', #20535, 11.00000000000000000 ) ;
#59318=EDGE_CURVE ( 'NONE', #55261, #1258, #55158, .T. ) ;
#59319=VECTOR ( 'NONE', #46556, 1000.000000000000000 ) ;
#59330=EDGE_CURVE ( 'NONE', #34549, #26676, #51294, .T. ) ;
#59338=EDGE_CURVE ( 'NONE', #55857, #17257, #49998, .T. ) ;
#59479=AXIS2_PLACEMENT_3D ( 'NONE', #62867, #37789, #18779 ) ;
#59644=STYLED_ITEM('',(#63698),#29015);
#59804=CARTESIAN_POINT ( 'NONE',  ( 75.00000000000001421, 0.000000000000000000, -9.000000000000001776 ) ) ;
#59864=CARTESIAN_POINT ( 'NONE',  ( 6.324555320336756381, 15.00000000000000000, -9.000000000000001776 ) ) ;
#59872=DIRECTION ( 'NONE',  ( -0.000000000000000000, 1.000000000000000000, -0.000000000000000000 ) ) ;
#59988=DIRECTION ( 'NONE',  ( 7.709882115452476194E-16, 0.000000000000000000, -1.000000000000000000 ) ) ;
#60299=ORIENTED_EDGE ( 'NONE', *, *, #6272, .F. ) ;
#60332=EDGE_LOOP ( 'NONE', ( #58204, #12975, #4801, #13856, #15836, #51877, #13670, #39449, #21440, #19765, #9872, #21287, #5688, #60299, #14074, #36159, #25136 ) ) ;
#60385=ORIENTED_EDGE ( 'NONE', *, *, #15761, .T. ) ;
#60400=CARTESIAN_POINT ( 'NONE',  ( -6.324555320336756381, 15.00000000000000000, -9.000000000000001776 ) ) ;
#60681=CARTESIAN_POINT ( 'NONE',  ( 75.00000000000000000, 15.00000000000000000, 8.999999999999998224 ) ) ;
#60854=EDGE_LOOP ( 'NONE', ( #57732, #57133, #54440, #26184 ) ) ;
#60870=ORIENTED_EDGE ( 'NONE', *, *, #61030, .T. ) ;
#61030=EDGE_CURVE ( 'NONE', #19898, #61397, #49108, .T. ) ;
#61061=( NAMED_UNIT ( * ) SI_UNIT ( $, .STERADIAN. ) SOLID_ANGLE_UNIT ( ) );
#61124=LINE ( 'NONE', #3217, #15006 ) ;
#61197=FACE_BOUND ( 'NONE', #25545, .T. ) ;
#61397=VERTEX_POINT ( 'NONE', #43316 ) ;
#61454=CARTESIAN_POINT ( 'NONE',  ( 75.00000000000002842, 0.000000000000000000, -5.000000000000000000 ) ) ;
#61499=AXIS2_PLACEMENT_3D ( 'NONE', #21202, #46601, #23028 ) ;
#61891=PLANE ( 'NONE',  #16955 ) ;
#61937=DIRECTION ( 'NONE',  ( 0.000000000000000000, 0.000000000000000000, 1.000000000000000000 ) ) ;
#61948=CARTESIAN_POINT ( 'NONE',  ( 75.00000000000002842, 0.000000000000000000, 5.000000000000000000 ) ) ;
#61961=EDGE_LOOP ( 'NONE', ( #17440, #17325, #32022, #14661, #57371, #13300, #30594, #7954, #19188, #53558, #24247, #10109, #33143, #43466, #14808, #40715, #52897 ) ) ;
#62021=EDGE_CURVE ( 'NONE', #19898, #16398, #22384, .T. ) ;
#62039=ORIENTED_EDGE ( 'NONE', *, *, #46867, .T. ) ;
#62054=AXIS2_PLACEMENT_3D ( 'NONE', #29765, #35889, #30086 ) ;
#62200=CARTESIAN_POINT ( 'NONE',  ( 0.000000000000000000, 0.000000000000000000, 0.000000000000000000 ) ) ;
#62204=DIRECTION ( 'NONE',  ( 1.000000000000000000, 0.000000000000000000, -7.709882115452477180E-16 ) ) ;
#62260=CARTESIAN_POINT ( 'NONE',  ( -75.00000000000002842, 15.00000000000000000, 5.000000000000000000 ) ) ;
#62656=DIRECTION ( 'NONE',  ( -0.000000000000000000, 0.000000000000000000, 1.000000000000000000 ) ) ;
#62743=VECTOR ( 'NONE', #37434, 1000.000000000000000 ) ;
#62867=CARTESIAN_POINT ( 'NONE',  ( -75.00000000000002842, 15.00000000000000000, 5.000000000000000000 ) ) ;
#62893=CARTESIAN_POINT ( 'NONE',  ( 75.00000000000000000, 0.000000000000000000, 8.999999999999998224 ) ) ;
#62939=DIRECTION ( 'NONE',  ( -1.000000000000000000, -0.000000000000000000, -0.000000000000000000 ) ) ;
#63075=PRODUCT_DEFINITION_CONTEXT ( 'detailed design', #48689, 'design' ) ;
#63097=CARTESIAN_POINT ( 'NONE',  ( -75.00000000000001421, 15.00000000000000000, -9.000000000000001776 ) ) ;
#63171=EDGE_CURVE ( 'NONE', #35107, #56115, #54719, .T. ) ;
#63520=PLANE ( 'NONE',  #35824 ) ;
#63524=UNCERTAINTY_MEASURE_WITH_UNIT (LENGTH_MEASURE( 1.000000000000000082E-05 ), #59255, 'distance_accuracy_value', 'NONE');
#63692=COLOUR_RGB('Light Blue',0.38,0.62,0.78);
#63693=FILL_AREA_STYLE_COLOUR('',#63692);
#63694=FILL_AREA_STYLE('',(#63693));
#63695=SURFACE_STYLE_FILL_AREA(#63694);
#63696=SURFACE_SIDE_STYLE('',(#63695));
#63697=SURFACE_STYLE_USAGE(.BOTH.,#63696);
#63698=PRESENTATION_STYLE_ASSIGNMENT((#63697));
ENDSEC;
END-ISO-10303-21;
